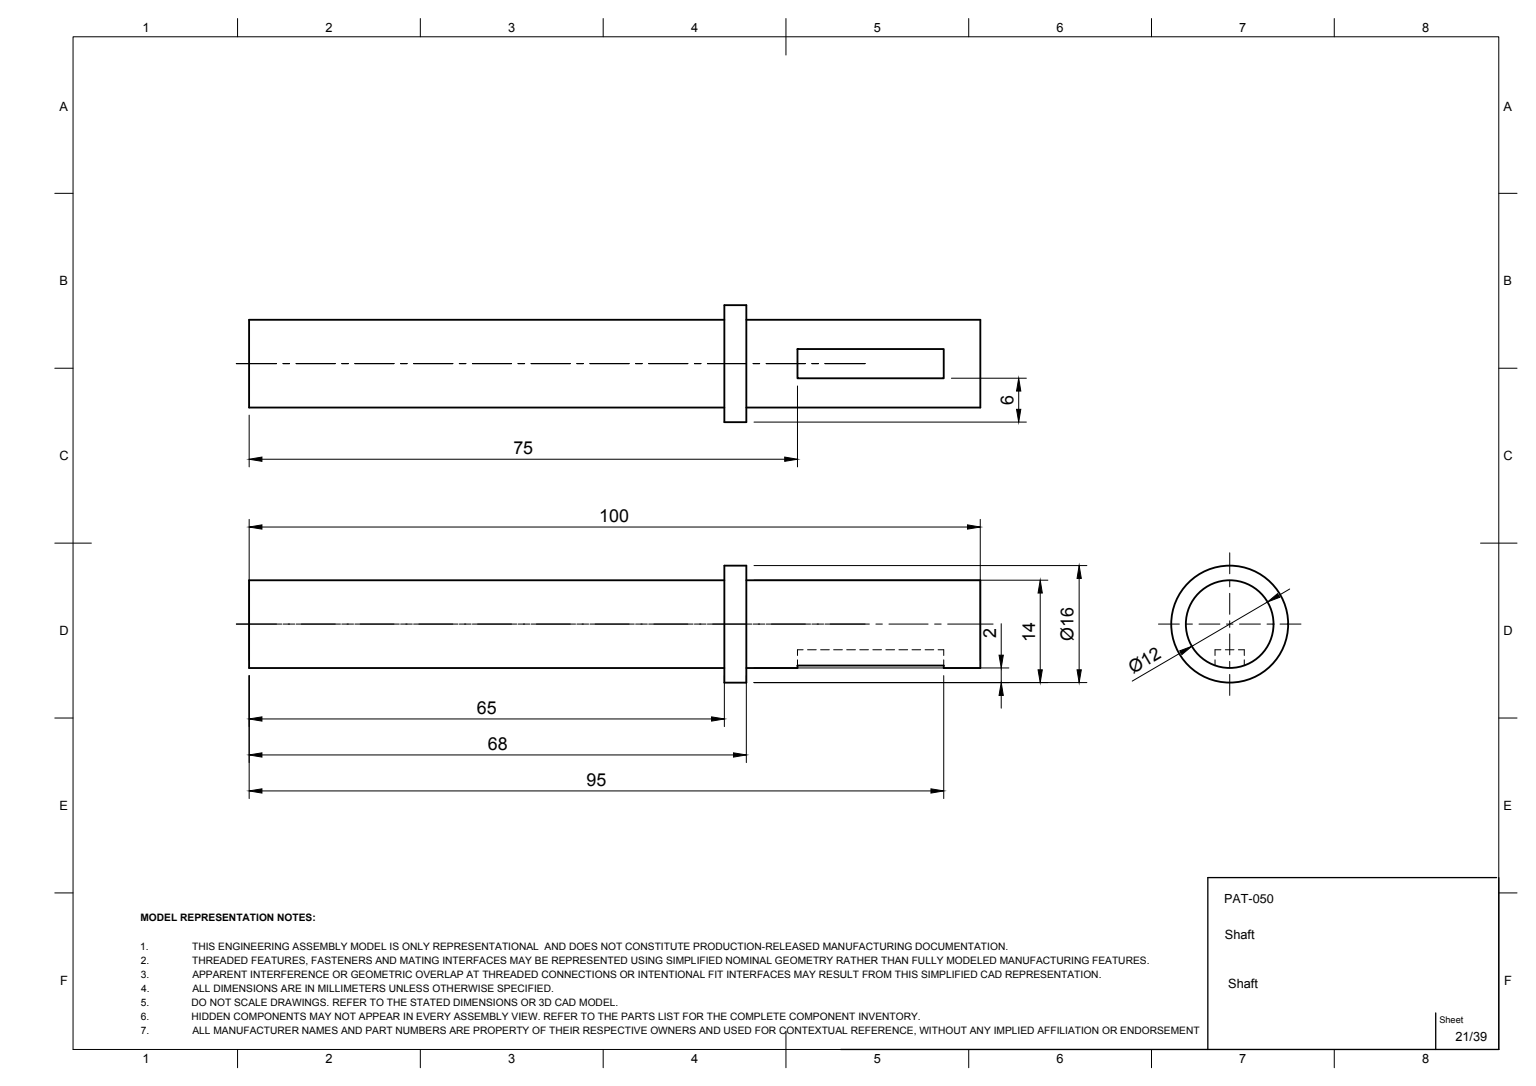
ISO-10303-21;
HEADER;
/* Generated by software containing ST-Developer
 * from STEP Tools, Inc. (www.steptools.com) 
 */

FILE_DESCRIPTION(
/* description */ ('Hand wheel with handle and shaft collar'),
/* implementation_level */ '2;1');

FILE_NAME(
/* name */ 'Shaft.step',
/* time_stamp */ '2026-10-28T03:23:19-07:00',
/* author */ (''),
/* organization */ (''),
/* preprocessor_version */ 'ST-DEVELOPER v20.2',
/* originating_system */ 'Autodesk Translation Framework v15.17.0.0',
/* authorisation */ '');

FILE_SCHEMA (('AUTOMOTIVE_DESIGN { 1 0 10303 214 3 1 1 }'));
ENDSEC;

DATA;
#10=MECHANICAL_DESIGN_GEOMETRIC_PRESENTATION_REPRESENTATION('',(#416),#10510);
#345=SHAPE_REPRESENTATION_RELATIONSHIP('SRR','None',#10663,#377);
#377=ADVANCED_BREP_SHAPE_REPRESENTATION('',(#462),#10490);
#416=STYLED_ITEM('',(#10908),#462);
#462=MANIFOLD_SOLID_BREP('Body1',#5316);
#548=FACE_BOUND('',#1283,.T.);
#549=FACE_BOUND('',#1285,.T.);
#550=FACE_BOUND('',#1288,.T.);
#663=PLANE('',#5992);
#664=PLANE('',#5993);
#665=PLANE('',#5995);
#666=PLANE('',#5996);
#667=PLANE('',#5997);
#668=PLANE('',#5999);
#669=PLANE('',#6002);
#670=PLANE('',#6010);
#671=PLANE('',#6011);
#896=FACE_OUTER_BOUND('',#1277,.T.);
#897=FACE_OUTER_BOUND('',#1278,.T.);
#898=FACE_OUTER_BOUND('',#1279,.T.);
#899=FACE_OUTER_BOUND('',#1280,.T.);
#900=FACE_OUTER_BOUND('',#1281,.T.);
#901=FACE_OUTER_BOUND('',#1282,.T.);
#902=FACE_OUTER_BOUND('',#1284,.T.);
#903=FACE_OUTER_BOUND('',#1286,.T.);
#904=FACE_OUTER_BOUND('',#1287,.T.);
#905=FACE_OUTER_BOUND('',#1289,.T.);
#906=FACE_OUTER_BOUND('',#1290,.T.);
#907=FACE_OUTER_BOUND('',#1291,.T.);
#1277=EDGE_LOOP('',(#4121,#4122,#4123,#4124));
#1278=EDGE_LOOP('',(#4125,#4126,#4127,#4128));
#1279=EDGE_LOOP('',(#4129,#4130,#4131,#4132));
#1280=EDGE_LOOP('',(#4133,#4134,#4135,#4136));
#1281=EDGE_LOOP('',(#4137,#4138,#4139,#4140));
#1282=EDGE_LOOP('',(#4141));
#1283=EDGE_LOOP('',(#4142));
#1284=EDGE_LOOP('',(#4143));
#1285=EDGE_LOOP('',(#4144));
#1286=EDGE_LOOP('',(#4145,#4146,#4147,#4148));
#1287=EDGE_LOOP('',(#4149,#4150,#4151,#4152));
#1288=EDGE_LOOP('',(#4153,#4154,#4155,#4156));
#1289=EDGE_LOOP('',(#4157,#4158,#4159,#4160));
#1290=EDGE_LOOP('',(#4161));
#1291=EDGE_LOOP('',(#4162));
#1643=LINE('',#9104,#1953);
#1644=LINE('',#9106,#1954);
#1645=LINE('',#9108,#1955);
#1646=LINE('',#9109,#1956);
#1647=LINE('',#9114,#1957);
#1648=LINE('',#9115,#1958);
#1649=LINE('',#9118,#1959);
#1650=LINE('',#9120,#1960);
#1651=LINE('',#9121,#1961);
#1652=LINE('',#9123,#1962);
#1653=LINE('',#9137,#1963);
#1654=LINE('',#9140,#1964);
#1655=LINE('',#9145,#1965);
#1953=VECTOR('',#7141,1.);
#1954=VECTOR('',#7142,1.);
#1955=VECTOR('',#7143,1.);
#1956=VECTOR('',#7144,1.);
#1957=VECTOR('',#7149,1.);
#1958=VECTOR('',#7150,1.);
#1959=VECTOR('',#7153,1.);
#1960=VECTOR('',#7154,1.);
#1961=VECTOR('',#7155,1.);
#1962=VECTOR('',#7158,1.);
#1963=VECTOR('',#7177,0.8);
#1964=VECTOR('',#7180,0.6);
#1965=VECTOR('',#7187,0.6);
#2271=CIRCLE('',#5994,0.6);
#2272=CIRCLE('',#5998,0.6);
#2273=CIRCLE('',#6000,0.8);
#2274=CIRCLE('',#6001,0.6);
#2275=CIRCLE('',#6003,0.8);
#2276=CIRCLE('',#6004,0.6);
#2277=CIRCLE('',#6007,0.6);
#2278=CIRCLE('',#6009,0.6);
#2639=VERTEX_POINT('',#9102);
#2640=VERTEX_POINT('',#9103);
#2641=VERTEX_POINT('',#9105);
#2642=VERTEX_POINT('',#9107);
#2643=VERTEX_POINT('',#9111);
#2644=VERTEX_POINT('',#9113);
#2645=VERTEX_POINT('',#9117);
#2646=VERTEX_POINT('',#9119);
#2647=VERTEX_POINT('',#9127);
#2648=VERTEX_POINT('',#9129);
#2649=VERTEX_POINT('',#9132);
#2650=VERTEX_POINT('',#9134);
#2651=VERTEX_POINT('',#9139);
#2652=VERTEX_POINT('',#9143);
#3178=EDGE_CURVE('',#2639,#2640,#1643,.T.);
#3179=EDGE_CURVE('',#2639,#2641,#1644,.T.);
#3180=EDGE_CURVE('',#2642,#2641,#1645,.T.);
#3181=EDGE_CURVE('',#2642,#2640,#1646,.T.);
#3182=EDGE_CURVE('',#2640,#2643,#2271,.T.);
#3183=EDGE_CURVE('',#2644,#2642,#1647,.T.);
#3184=EDGE_CURVE('',#2643,#2644,#1648,.T.);
#3185=EDGE_CURVE('',#2643,#2645,#1649,.T.);
#3186=EDGE_CURVE('',#2644,#2646,#1650,.T.);
#3187=EDGE_CURVE('',#2646,#2645,#1651,.T.);
#3188=EDGE_CURVE('',#2641,#2646,#1652,.T.);
#3189=EDGE_CURVE('',#2645,#2639,#2272,.T.);
#3190=EDGE_CURVE('',#2647,#2647,#2273,.T.);
#3191=EDGE_CURVE('',#2648,#2648,#2274,.T.);
#3192=EDGE_CURVE('',#2649,#2649,#2275,.T.);
#3193=EDGE_CURVE('',#2650,#2650,#2276,.T.);
#3194=EDGE_CURVE('',#2647,#2649,#1653,.T.);
#3195=EDGE_CURVE('',#2650,#2651,#1654,.T.);
#3196=EDGE_CURVE('',#2651,#2651,#2277,.T.);
#3197=EDGE_CURVE('',#2652,#2652,#2278,.T.);
#3198=EDGE_CURVE('',#2652,#2648,#1655,.T.);
#4121=ORIENTED_EDGE('',*,*,#3178,.F.);
#4122=ORIENTED_EDGE('',*,*,#3179,.T.);
#4123=ORIENTED_EDGE('',*,*,#3180,.F.);
#4124=ORIENTED_EDGE('',*,*,#3181,.T.);
#4125=ORIENTED_EDGE('',*,*,#3182,.F.);
#4126=ORIENTED_EDGE('',*,*,#3181,.F.);
#4127=ORIENTED_EDGE('',*,*,#3183,.F.);
#4128=ORIENTED_EDGE('',*,*,#3184,.F.);
#4129=ORIENTED_EDGE('',*,*,#3185,.F.);
#4130=ORIENTED_EDGE('',*,*,#3184,.T.);
#4131=ORIENTED_EDGE('',*,*,#3186,.T.);
#4132=ORIENTED_EDGE('',*,*,#3187,.T.);
#4133=ORIENTED_EDGE('',*,*,#3183,.T.);
#4134=ORIENTED_EDGE('',*,*,#3180,.T.);
#4135=ORIENTED_EDGE('',*,*,#3188,.T.);
#4136=ORIENTED_EDGE('',*,*,#3186,.F.);
#4137=ORIENTED_EDGE('',*,*,#3189,.F.);
#4138=ORIENTED_EDGE('',*,*,#3187,.F.);
#4139=ORIENTED_EDGE('',*,*,#3188,.F.);
#4140=ORIENTED_EDGE('',*,*,#3179,.F.);
#4141=ORIENTED_EDGE('',*,*,#3190,.T.);
#4142=ORIENTED_EDGE('',*,*,#3191,.F.);
#4143=ORIENTED_EDGE('',*,*,#3192,.F.);
#4144=ORIENTED_EDGE('',*,*,#3193,.F.);
#4145=ORIENTED_EDGE('',*,*,#3190,.F.);
#4146=ORIENTED_EDGE('',*,*,#3194,.T.);
#4147=ORIENTED_EDGE('',*,*,#3192,.T.);
#4148=ORIENTED_EDGE('',*,*,#3194,.F.);
#4149=ORIENTED_EDGE('',*,*,#3193,.T.);
#4150=ORIENTED_EDGE('',*,*,#3195,.T.);
#4151=ORIENTED_EDGE('',*,*,#3196,.T.);
#4152=ORIENTED_EDGE('',*,*,#3195,.F.);
#4153=ORIENTED_EDGE('',*,*,#3185,.T.);
#4154=ORIENTED_EDGE('',*,*,#3189,.T.);
#4155=ORIENTED_EDGE('',*,*,#3178,.T.);
#4156=ORIENTED_EDGE('',*,*,#3182,.T.);
#4157=ORIENTED_EDGE('',*,*,#3197,.F.);
#4158=ORIENTED_EDGE('',*,*,#3198,.T.);
#4159=ORIENTED_EDGE('',*,*,#3191,.T.);
#4160=ORIENTED_EDGE('',*,*,#3198,.F.);
#4161=ORIENTED_EDGE('',*,*,#3197,.T.);
#4162=ORIENTED_EDGE('',*,*,#3196,.F.);
#4924=CYLINDRICAL_SURFACE('',#6005,0.8);
#4925=CYLINDRICAL_SURFACE('',#6006,0.6);
#4926=CYLINDRICAL_SURFACE('',#6008,0.6);
#5108=ADVANCED_FACE('',(#896),#663,.F.);
#5109=ADVANCED_FACE('',(#897),#664,.T.);
#5110=ADVANCED_FACE('',(#898),#665,.F.);
#5111=ADVANCED_FACE('',(#899),#666,.F.);
#5112=ADVANCED_FACE('',(#900),#667,.F.);
#5113=ADVANCED_FACE('',(#901,#548),#668,.T.);
#5114=ADVANCED_FACE('',(#902,#549),#669,.F.);
#5115=ADVANCED_FACE('',(#903),#4924,.T.);
#5116=ADVANCED_FACE('',(#904,#550),#4925,.T.);
#5117=ADVANCED_FACE('',(#905),#4926,.T.);
#5118=ADVANCED_FACE('',(#906),#670,.T.);
#5119=ADVANCED_FACE('',(#907),#671,.F.);
#5316=CLOSED_SHELL('',(#5108,#5109,#5110,#5111,#5112,#5113,#5114,#5115,
#5116,#5117,#5118,#5119));
#5991=AXIS2_PLACEMENT_3D('',#9100,#7137,#7138);
#5992=AXIS2_PLACEMENT_3D('',#9101,#7139,#7140);
#5993=AXIS2_PLACEMENT_3D('',#9110,#7145,#7146);
#5994=AXIS2_PLACEMENT_3D('',#9112,#7147,#7148);
#5995=AXIS2_PLACEMENT_3D('',#9116,#7151,#7152);
#5996=AXIS2_PLACEMENT_3D('',#9122,#7156,#7157);
#5997=AXIS2_PLACEMENT_3D('',#9124,#7159,#7160);
#5998=AXIS2_PLACEMENT_3D('',#9125,#7161,#7162);
#5999=AXIS2_PLACEMENT_3D('',#9126,#7163,#7164);
#6000=AXIS2_PLACEMENT_3D('',#9128,#7165,#7166);
#6001=AXIS2_PLACEMENT_3D('',#9130,#7167,#7168);
#6002=AXIS2_PLACEMENT_3D('',#9131,#7169,#7170);
#6003=AXIS2_PLACEMENT_3D('',#9133,#7171,#7172);
#6004=AXIS2_PLACEMENT_3D('',#9135,#7173,#7174);
#6005=AXIS2_PLACEMENT_3D('',#9136,#7175,#7176);
#6006=AXIS2_PLACEMENT_3D('',#9138,#7178,#7179);
#6007=AXIS2_PLACEMENT_3D('',#9141,#7181,#7182);
#6008=AXIS2_PLACEMENT_3D('',#9142,#7183,#7184);
#6009=AXIS2_PLACEMENT_3D('',#9144,#7185,#7186);
#6010=AXIS2_PLACEMENT_3D('',#9146,#7188,#7189);
#6011=AXIS2_PLACEMENT_3D('',#9147,#7190,#7191);
#7137=DIRECTION('axis',(0.,0.,1.));
#7138=DIRECTION('refdir',(1.,0.,0.));
#7139=DIRECTION('center_axis',(-1.,0.,0.));
#7140=DIRECTION('ref_axis',(0.,0.,1.));
#7141=DIRECTION('',(0.,-1.,0.));
#7142=DIRECTION('',(0.,0.,1.));
#7143=DIRECTION('',(0.,1.,0.));
#7144=DIRECTION('',(0.,0.,-1.));
#7145=DIRECTION('center_axis',(0.,1.,0.));
#7146=DIRECTION('ref_axis',(1.,0.,0.));
#7147=DIRECTION('center_axis',(0.,-1.,0.));
#7148=DIRECTION('ref_axis',(1.,0.,0.));
#7149=DIRECTION('',(-1.,0.,0.));
#7150=DIRECTION('',(0.,0.,1.));
#7151=DIRECTION('center_axis',(1.,0.,0.));
#7152=DIRECTION('ref_axis',(0.,0.,-1.));
#7153=DIRECTION('',(0.,1.,0.));
#7154=DIRECTION('',(0.,1.,0.));
#7155=DIRECTION('',(0.,0.,-1.));
#7156=DIRECTION('center_axis',(0.,0.,1.));
#7157=DIRECTION('ref_axis',(1.,0.,0.));
#7158=DIRECTION('',(1.,0.,0.));
#7159=DIRECTION('center_axis',(0.,1.,0.));
#7160=DIRECTION('ref_axis',(0.,0.,1.));
#7161=DIRECTION('center_axis',(0.,1.,0.));
#7162=DIRECTION('ref_axis',(1.,0.,0.));
#7163=DIRECTION('center_axis',(0.,1.,0.));
#7164=DIRECTION('ref_axis',(1.,0.,0.));
#7165=DIRECTION('center_axis',(0.,1.,0.));
#7166=DIRECTION('ref_axis',(1.,0.,0.));
#7167=DIRECTION('center_axis',(0.,1.,0.));
#7168=DIRECTION('ref_axis',(1.,0.,0.));
#7169=DIRECTION('center_axis',(0.,1.,0.));
#7170=DIRECTION('ref_axis',(1.,0.,0.));
#7171=DIRECTION('center_axis',(0.,1.,0.));
#7172=DIRECTION('ref_axis',(1.,0.,0.));
#7173=DIRECTION('center_axis',(0.,-1.,0.));
#7174=DIRECTION('ref_axis',(1.,0.,0.));
#7175=DIRECTION('center_axis',(0.,1.,0.));
#7176=DIRECTION('ref_axis',(1.,0.,0.));
#7177=DIRECTION('',(0.,-1.,0.));
#7178=DIRECTION('center_axis',(0.,1.,0.));
#7179=DIRECTION('ref_axis',(1.,0.,0.));
#7180=DIRECTION('',(0.,-1.,0.));
#7181=DIRECTION('center_axis',(0.,1.,0.));
#7182=DIRECTION('ref_axis',(1.,0.,0.));
#7183=DIRECTION('center_axis',(0.,1.,0.));
#7184=DIRECTION('ref_axis',(1.,0.,0.));
#7185=DIRECTION('center_axis',(0.,1.,0.));
#7186=DIRECTION('ref_axis',(1.,0.,0.));
#7187=DIRECTION('',(0.,-1.,0.));
#7188=DIRECTION('center_axis',(0.,1.,0.));
#7189=DIRECTION('ref_axis',(1.,0.,0.));
#7190=DIRECTION('center_axis',(0.,1.,0.));
#7191=DIRECTION('ref_axis',(1.,0.,0.));
#9100=CARTESIAN_POINT('',(0.,0.,0.));
#9101=CARTESIAN_POINT('Origin',(-0.2,-3.5,9.3));
#9102=CARTESIAN_POINT('',(-0.2,-1.5,9.43431457505076));
#9103=CARTESIAN_POINT('',(-0.2,-3.5,9.43431457505076));
#9104=CARTESIAN_POINT('',(-0.2,-4.,9.43431457505076));
#9105=CARTESIAN_POINT('',(-0.2,-1.5,9.65));
#9106=CARTESIAN_POINT('',(-0.2,-1.5,9.65));
#9107=CARTESIAN_POINT('',(-0.2,-3.5,9.65));
#9108=CARTESIAN_POINT('',(-0.2,-3.5,9.65));
#9109=CARTESIAN_POINT('',(-0.2,-3.5,9.65));
#9110=CARTESIAN_POINT('Origin',(0.,-3.5,9.475));
#9111=CARTESIAN_POINT('',(0.2,-3.5,9.43431457505076));
#9112=CARTESIAN_POINT('Origin',(0.,-3.5,10.));
#9113=CARTESIAN_POINT('',(0.2,-3.5,9.65));
#9114=CARTESIAN_POINT('',(0.2,-3.5,9.65));
#9115=CARTESIAN_POINT('',(0.2,-3.5,9.3));
#9116=CARTESIAN_POINT('Origin',(0.2,-3.5,9.65));
#9117=CARTESIAN_POINT('',(0.2,-1.5,9.43431457505076));
#9118=CARTESIAN_POINT('',(0.2,-4.,9.43431457505076));
#9119=CARTESIAN_POINT('',(0.2,-1.5,9.65));
#9120=CARTESIAN_POINT('',(0.2,-3.5,9.65));
#9121=CARTESIAN_POINT('',(0.2,-1.5,9.3));
#9122=CARTESIAN_POINT('Origin',(-0.2,-3.5,9.65));
#9123=CARTESIAN_POINT('',(0.2,-1.5,9.65));
#9124=CARTESIAN_POINT('Origin',(0.,-1.5,9.475));
#9125=CARTESIAN_POINT('Origin',(0.,-1.5,10.));
#9126=CARTESIAN_POINT('Origin',(0.,-0.5,10.));
#9127=CARTESIAN_POINT('',(-0.8,-0.5,10.));
#9128=CARTESIAN_POINT('Origin',(0.,-0.5,10.));
#9129=CARTESIAN_POINT('',(-0.6,-0.5,10.));
#9130=CARTESIAN_POINT('Origin',(0.,-0.5,10.));
#9131=CARTESIAN_POINT('Origin',(0.,-0.8,10.));
#9132=CARTESIAN_POINT('',(-0.8,-0.8,10.));
#9133=CARTESIAN_POINT('Origin',(0.,-0.8,10.));
#9134=CARTESIAN_POINT('',(-0.6,-0.8,10.));
#9135=CARTESIAN_POINT('Origin',(0.,-0.8,10.));
#9136=CARTESIAN_POINT('Origin',(0.,-0.8,10.));
#9137=CARTESIAN_POINT('',(-0.8,-0.8,10.));
#9138=CARTESIAN_POINT('Origin',(0.,-4.,10.));
#9139=CARTESIAN_POINT('',(-0.6,-4.,10.));
#9140=CARTESIAN_POINT('',(-0.6,-4.,10.));
#9141=CARTESIAN_POINT('Origin',(0.,-4.,10.));
#9142=CARTESIAN_POINT('Origin',(0.,-4.,10.));
#9143=CARTESIAN_POINT('',(-0.6,6.,10.));
#9144=CARTESIAN_POINT('Origin',(0.,6.,10.));
#9145=CARTESIAN_POINT('',(-0.6,-4.,10.));
#9146=CARTESIAN_POINT('Origin',(0.,6.,10.));
#9147=CARTESIAN_POINT('Origin',(0.,-4.,10.));
#10451=UNCERTAINTY_MEASURE_WITH_UNIT(LENGTH_MEASURE(0.001),#10511,
'DISTANCE_ACCURACY_VALUE',
'Maximum model space distance between geometric entities at asserted c
onnectivities');
#10471=UNCERTAINTY_MEASURE_WITH_UNIT(LENGTH_MEASURE(0.001),#10511,
'DISTANCE_ACCURACY_VALUE',
'Maximum model space distance between geometric entities at asserted c
onnectivities');
#10490=(
GEOMETRIC_REPRESENTATION_CONTEXT(3)
GLOBAL_UNCERTAINTY_ASSIGNED_CONTEXT((#10451))
GLOBAL_UNIT_ASSIGNED_CONTEXT((#10511,#10513,#10514))
REPRESENTATION_CONTEXT('','3D')
);
#10510=(
GEOMETRIC_REPRESENTATION_CONTEXT(3)
GLOBAL_UNCERTAINTY_ASSIGNED_CONTEXT((#10471))
GLOBAL_UNIT_ASSIGNED_CONTEXT((#10511,#10513,#10514))
REPRESENTATION_CONTEXT('','3D')
);
#10511=(
LENGTH_UNIT()
NAMED_UNIT(*)
SI_UNIT(.CENTI.,.METRE.)
);
#10513=(
NAMED_UNIT(*)
PLANE_ANGLE_UNIT()
SI_UNIT($,.RADIAN.)
);
#10514=(
NAMED_UNIT(*)
SI_UNIT($,.STERADIAN.)
SOLID_ANGLE_UNIT()
);
#10533=SHAPE_DEFINITION_REPRESENTATION(#10576,#10663);
#10576=PRODUCT_DEFINITION_SHAPE('',$,#10702);
#10663=SHAPE_REPRESENTATION('',(#5991),#10490);
#10683=PRODUCT_DEFINITION_CONTEXT('part definition',#10799,'design');
#10702=PRODUCT_DEFINITION('Shaft','Shaft',#10740,#10683);
#10740=PRODUCT_DEFINITION_FORMATION('',$,#10819);
#10799=APPLICATION_CONTEXT(
'Core Data for Automotive Mechanical Design Process');
#10800=PRODUCT_CONTEXT('part definition',#10799,'mechanical');
#10819=PRODUCT('Shaft','Shaft','Shaft',(#10800));
#10902=COLOUR_RGB('Grey',0.48,0.52,0.57);
#10903=FILL_AREA_STYLE_COLOUR('',#10902);
#10904=FILL_AREA_STYLE('',(#10903));
#10905=SURFACE_STYLE_FILL_AREA(#10904);
#10906=SURFACE_SIDE_STYLE('',(#10905));
#10907=SURFACE_STYLE_USAGE(.BOTH.,#10906);
#10908=PRESENTATION_STYLE_ASSIGNMENT((#10907));
ENDSEC;
END-ISO-10303-21;
